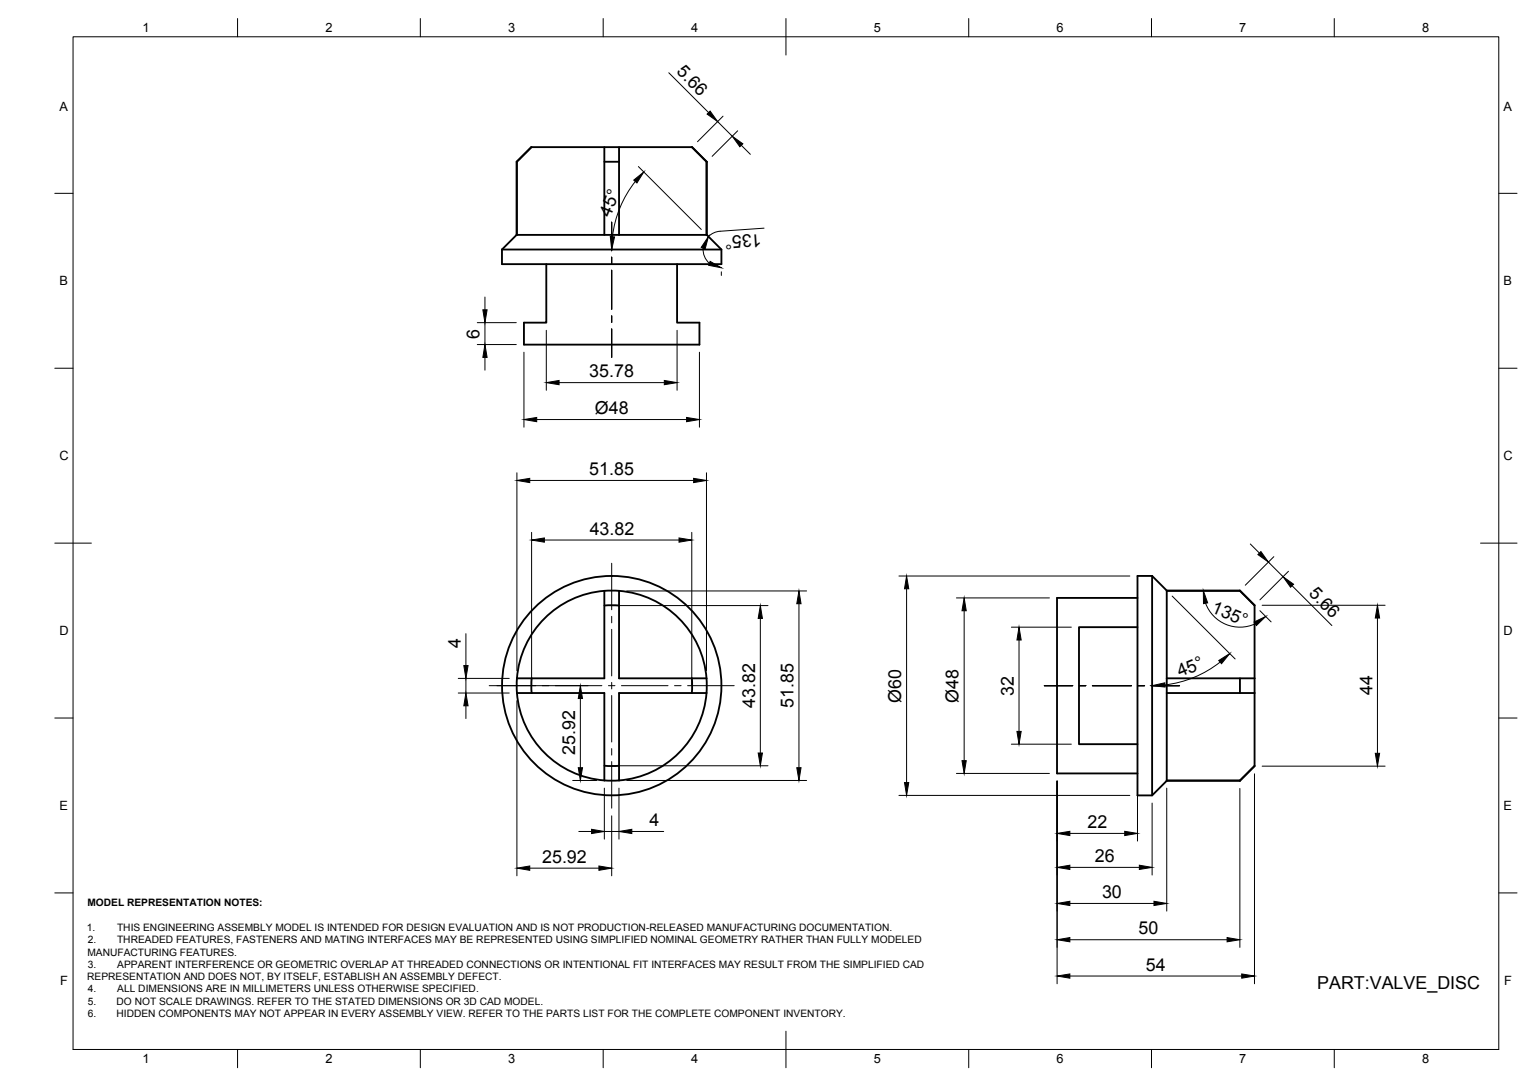
ISO-10303-21;
HEADER;
/* Generated by software containing ST-Developer
 * from STEP Tools, Inc. (www.steptools.com) 
 */

FILE_DESCRIPTION(
/* description */ (''),
/* implementation_level */ '2;1');

FILE_NAME(
/* name */ 'VALVE_DISC.step',
/* time_stamp */ '2026-10-04T02:10:06-07:00',
/* author */ (''),
/* organization */ (''),
/* preprocessor_version */ 'ST-DEVELOPER v20.2',
/* originating_system */ 'Autodesk Translation Framework v15.15.0.0',
/* authorisation */ '');

FILE_SCHEMA (('AUTOMOTIVE_DESIGN { 1 0 10303 214 3 1 1 }'));
ENDSEC;

DATA;
#10=MECHANICAL_DESIGN_GEOMETRIC_PRESENTATION_REPRESENTATION('',(#142),#9668);
#75=(
BOUNDED_CURVE()
B_SPLINE_CURVE(2,(#6291,#6292,#6293),.UNSPECIFIED.,.F.,.F.)
B_SPLINE_CURVE_WITH_KNOTS((3,3),(-0.968089558975317,-0.208236182755166),
 .UNSPECIFIED.)
CURVE()
GEOMETRIC_REPRESENTATION_ITEM()
RATIONAL_B_SPLINE_CURVE((1.03202593839996,1.02394290093172,1.00881846372195))
REPRESENTATION_ITEM('')
);
#76=(
BOUNDED_CURVE()
B_SPLINE_CURVE(2,(#6302,#6303,#6304),.UNSPECIFIED.,.F.,.F.)
B_SPLINE_CURVE_WITH_KNOTS((3,3),(-3.47246065490362,-2.71260727868867),
 .UNSPECIFIED.)
CURVE()
GEOMETRIC_REPRESENTATION_ITEM()
RATIONAL_B_SPLINE_CURVE((1.00881846372215,1.02394290093178,1.03202593839996))
REPRESENTATION_ITEM('')
);
#77=(
BOUNDED_CURVE()
B_SPLINE_CURVE(2,(#6312,#6313,#6314),.UNSPECIFIED.,.F.,.F.)
B_SPLINE_CURVE_WITH_KNOTS((3,3),(-3.47246065490362,-2.71260727868867),
 .UNSPECIFIED.)
CURVE()
GEOMETRIC_REPRESENTATION_ITEM()
RATIONAL_B_SPLINE_CURVE((1.00881846372215,1.02394290093178,1.03202593839996))
REPRESENTATION_ITEM('')
);
#78=(
BOUNDED_CURVE()
B_SPLINE_CURVE(2,(#6321,#6322,#6323),.UNSPECIFIED.,.F.,.F.)
B_SPLINE_CURVE_WITH_KNOTS((3,3),(-0.968089558975317,-0.208236182755166),
 .UNSPECIFIED.)
CURVE()
GEOMETRIC_REPRESENTATION_ITEM()
RATIONAL_B_SPLINE_CURVE((1.03202593839996,1.02394290093172,1.00881846372195))
REPRESENTATION_ITEM('')
);
#79=(
BOUNDED_CURVE()
B_SPLINE_CURVE(2,(#6399,#6400,#6401),.UNSPECIFIED.,.F.,.F.)
B_SPLINE_CURVE_WITH_KNOTS((3,3),(-3.47246065490413,-2.71260727868925),
 .UNSPECIFIED.)
CURVE()
GEOMETRIC_REPRESENTATION_ITEM()
RATIONAL_B_SPLINE_CURVE((1.00881846372252,1.0239429009328,1.03202593840134))
REPRESENTATION_ITEM('')
);
#80=(
BOUNDED_CURVE()
B_SPLINE_CURVE(2,(#6406,#6407,#6408),.UNSPECIFIED.,.F.,.F.)
B_SPLINE_CURVE_WITH_KNOTS((3,3),(-0.968089559028266,-0.20823618276597),
 .UNSPECIFIED.)
CURVE()
GEOMETRIC_REPRESENTATION_ITEM()
RATIONAL_B_SPLINE_CURVE((1.03202593842995,1.02394290095447,1.00881846373032))
REPRESENTATION_ITEM('')
);
#81=(
BOUNDED_CURVE()
B_SPLINE_CURVE(2,(#6413,#6414,#6415),.UNSPECIFIED.,.F.,.F.)
B_SPLINE_CURVE_WITH_KNOTS((3,3),(-3.47246065490413,-2.71260727868925),
 .UNSPECIFIED.)
CURVE()
GEOMETRIC_REPRESENTATION_ITEM()
RATIONAL_B_SPLINE_CURVE((1.00881846372251,1.0239429009328,1.03202593840134))
REPRESENTATION_ITEM('')
);
#82=(
BOUNDED_CURVE()
B_SPLINE_CURVE(2,(#6420,#6421,#6422),.UNSPECIFIED.,.F.,.F.)
B_SPLINE_CURVE_WITH_KNOTS((3,3),(-0.968089559028514,-0.208236182766157),
 .UNSPECIFIED.)
CURVE()
GEOMETRIC_REPRESENTATION_ITEM()
RATIONAL_B_SPLINE_CURVE((1.03202593842948,1.02394290095412,1.0088184637302))
REPRESENTATION_ITEM('')
);
#120=SHAPE_REPRESENTATION_RELATIONSHIP('SRR','None',#9713,#131);
#131=ADVANCED_BREP_SHAPE_REPRESENTATION('',(#153),#9658);
#142=STYLED_ITEM('',(#9775),#153);
#153=MANIFOLD_SOLID_BREP('Body1',#3882);
#165=CONICAL_SURFACE('',#4162,26.,0.785398163397448);
#166=CONICAL_SURFACE('',#4190,22.,0.785398163397446);
#167=CONICAL_SURFACE('',#4191,22.,0.785398163397446);
#168=CONICAL_SURFACE('',#4192,22.,0.785398163397446);
#169=CONICAL_SURFACE('',#4193,22.,0.785398163397446);
#229=FACE_BOUND('',#1124,.T.);
#230=FACE_BOUND('',#1127,.T.);
#231=FACE_BOUND('',#1128,.T.);
#232=FACE_BOUND('',#1133,.T.);
#281=PLANE('',#4136);
#282=PLANE('',#4138);
#283=PLANE('',#4140);
#284=PLANE('',#4142);
#285=PLANE('',#4144);
#286=PLANE('',#4145);
#287=PLANE('',#4146);
#288=PLANE('',#4147);
#289=PLANE('',#4148);
#290=PLANE('',#4157);
#291=PLANE('',#4168);
#292=PLANE('',#4169);
#293=PLANE('',#4171);
#294=PLANE('',#4177);
#295=PLANE('',#4182);
#296=PLANE('',#4183);
#297=PLANE('',#4186);
#298=PLANE('',#4187);
#406=LINE('',#6264,#597);
#407=LINE('',#6265,#598);
#408=LINE('',#6269,#599);
#409=LINE('',#6271,#600);
#410=LINE('',#6276,#601);
#411=LINE('',#6278,#602);
#412=LINE('',#6285,#603);
#413=LINE('',#6286,#604);
#414=LINE('',#6289,#605);
#415=LINE('',#6295,#606);
#416=LINE('',#6296,#607);
#417=LINE('',#6300,#608);
#418=LINE('',#6305,#609);
#419=LINE('',#6306,#610);
#420=LINE('',#6310,#611);
#421=LINE('',#6315,#612);
#422=LINE('',#6316,#613);
#423=LINE('',#6319,#614);
#424=LINE('',#6325,#615);
#425=LINE('',#6326,#616);
#426=LINE('',#6335,#617);
#427=LINE('',#6338,#618);
#428=LINE('',#6342,#619);
#429=LINE('',#6346,#620);
#430=LINE('',#6350,#621);
#431=LINE('',#6355,#622);
#432=LINE('',#6356,#623);
#433=LINE('',#6362,#624);
#434=LINE('',#6365,#625);
#435=LINE('',#6372,#626);
#436=LINE('',#6374,#627);
#437=LINE('',#6379,#628);
#438=LINE('',#6386,#629);
#439=LINE('',#6389,#630);
#440=LINE('',#6392,#631);
#441=LINE('',#6395,#632);
#442=LINE('',#6402,#633);
#443=LINE('',#6405,#634);
#444=LINE('',#6416,#635);
#445=LINE('',#6419,#636);
#597=VECTOR('',#4752,23.9229627936314);
#598=VECTOR('',#4753,23.9229627936314);
#599=VECTOR('',#4756,23.9229627936314);
#600=VECTOR('',#4757,23.9229627936314);
#601=VECTOR('',#4762,23.9229627936314);
#602=VECTOR('',#4763,23.9229627936314);
#603=VECTOR('',#4770,23.9229627936314);
#604=VECTOR('',#4771,23.9229627936314);
#605=VECTOR('',#4774,20.);
#606=VECTOR('',#4775,19.9089023002066);
#607=VECTOR('',#4776,24.);
#608=VECTOR('',#4779,19.9089023002066);
#609=VECTOR('',#4780,20.);
#610=VECTOR('',#4781,24.);
#611=VECTOR('',#4784,19.9089023002066);
#612=VECTOR('',#4785,20.);
#613=VECTOR('',#4786,24.);
#614=VECTOR('',#4789,20.);
#615=VECTOR('',#4790,19.9089023002066);
#616=VECTOR('',#4791,24.);
#617=VECTOR('',#4800,16.);
#618=VECTOR('',#4803,24.);
#619=VECTOR('',#4806,16.);
#620=VECTOR('',#4809,16.);
#621=VECTOR('',#4812,16.);
#622=VECTOR('',#4819,35.7770876399966);
#623=VECTOR('',#4820,35.7770876399966);
#624=VECTOR('',#4827,30.);
#625=VECTOR('',#4830,26.);
#626=VECTOR('',#4843,35.7770876399966);
#627=VECTOR('',#4846,35.7770876399966);
#628=VECTOR('',#4853,11.);
#629=VECTOR('',#4864,19.9089023002066);
#630=VECTOR('',#4867,19.9089023002066);
#631=VECTOR('',#4870,19.9089023002066);
#632=VECTOR('',#4873,19.9089023002066);
#633=VECTOR('',#4878,20.);
#634=VECTOR('',#4881,20.);
#635=VECTOR('',#4888,20.);
#636=VECTOR('',#4891,20.);
#779=CYLINDRICAL_SURFACE('',#4151,24.);
#780=CYLINDRICAL_SURFACE('',#4159,30.);
#781=CYLINDRICAL_SURFACE('',#4172,11.);
#782=CYLINDRICAL_SURFACE('',#4173,26.);
#783=CYLINDRICAL_SURFACE('',#4175,26.);
#784=CYLINDRICAL_SURFACE('',#4184,26.);
#785=CYLINDRICAL_SURFACE('',#4188,26.);
#858=FACE_OUTER_BOUND('',#1115,.T.);
#859=FACE_OUTER_BOUND('',#1116,.T.);
#860=FACE_OUTER_BOUND('',#1117,.T.);
#861=FACE_OUTER_BOUND('',#1118,.T.);
#862=FACE_OUTER_BOUND('',#1119,.T.);
#863=FACE_OUTER_BOUND('',#1120,.T.);
#864=FACE_OUTER_BOUND('',#1121,.T.);
#865=FACE_OUTER_BOUND('',#1122,.T.);
#866=FACE_OUTER_BOUND('',#1123,.T.);
#867=FACE_OUTER_BOUND('',#1125,.T.);
#868=FACE_OUTER_BOUND('',#1126,.T.);
#869=FACE_OUTER_BOUND('',#1129,.T.);
#870=FACE_OUTER_BOUND('',#1130,.T.);
#871=FACE_OUTER_BOUND('',#1131,.T.);
#872=FACE_OUTER_BOUND('',#1132,.T.);
#873=FACE_OUTER_BOUND('',#1134,.T.);
#874=FACE_OUTER_BOUND('',#1135,.T.);
#875=FACE_OUTER_BOUND('',#1136,.T.);
#876=FACE_OUTER_BOUND('',#1137,.T.);
#877=FACE_OUTER_BOUND('',#1138,.T.);
#878=FACE_OUTER_BOUND('',#1139,.T.);
#879=FACE_OUTER_BOUND('',#1140,.T.);
#880=FACE_OUTER_BOUND('',#1141,.T.);
#881=FACE_OUTER_BOUND('',#1142,.T.);
#882=FACE_OUTER_BOUND('',#1143,.T.);
#883=FACE_OUTER_BOUND('',#1144,.T.);
#884=FACE_OUTER_BOUND('',#1145,.T.);
#885=FACE_OUTER_BOUND('',#1146,.T.);
#886=FACE_OUTER_BOUND('',#1147,.T.);
#887=FACE_OUTER_BOUND('',#1148,.T.);
#1115=EDGE_LOOP('',(#2781,#2782,#2783));
#1116=EDGE_LOOP('',(#2784,#2785,#2786));
#1117=EDGE_LOOP('',(#2787,#2788,#2789));
#1118=EDGE_LOOP('',(#2790,#2791,#2792));
#1119=EDGE_LOOP('',(#2793,#2794,#2795,#2796,#2797));
#1120=EDGE_LOOP('',(#2798,#2799,#2800,#2801,#2802));
#1121=EDGE_LOOP('',(#2803,#2804,#2805,#2806,#2807));
#1122=EDGE_LOOP('',(#2808,#2809,#2810,#2811,#2812));
#1123=EDGE_LOOP('',(#2813));
#1124=EDGE_LOOP('',(#2814));
#1125=EDGE_LOOP('',(#2815,#2816,#2817,#2818,#2819,#2820,#2821,#2822,#2823,
#2824,#2825,#2826));
#1126=EDGE_LOOP('',(#2827));
#1127=EDGE_LOOP('',(#2828,#2829));
#1128=EDGE_LOOP('',(#2830,#2831));
#1129=EDGE_LOOP('',(#2832,#2833,#2834,#2835,#2836));
#1130=EDGE_LOOP('',(#2837,#2838,#2839,#2840,#2841,#2842,#2843,#2844,#2845,
#2846,#2847,#2848,#2849));
#1131=EDGE_LOOP('',(#2850,#2851,#2852,#2853));
#1132=EDGE_LOOP('',(#2854,#2855,#2856,#2857,#2858));
#1133=EDGE_LOOP('',(#2859));
#1134=EDGE_LOOP('',(#2860,#2861,#2862,#2863));
#1135=EDGE_LOOP('',(#2864,#2865,#2866,#2867));
#1136=EDGE_LOOP('',(#2868,#2869,#2870,#2871));
#1137=EDGE_LOOP('',(#2872,#2873,#2874,#2875));
#1138=EDGE_LOOP('',(#2876,#2877,#2878,#2879,#2880,#2881,#2882,#2883,#2884,
#2885,#2886,#2887));
#1139=EDGE_LOOP('',(#2888,#2889,#2890,#2891,#2892));
#1140=EDGE_LOOP('',(#2893,#2894,#2895,#2896,#2897));
#1141=EDGE_LOOP('',(#2898,#2899,#2900,#2901,#2902));
#1142=EDGE_LOOP('',(#2903,#2904,#2905,#2906,#2907));
#1143=EDGE_LOOP('',(#2908,#2909,#2910,#2911,#2912));
#1144=EDGE_LOOP('',(#2913,#2914,#2915,#2916));
#1145=EDGE_LOOP('',(#2917,#2918,#2919,#2920));
#1146=EDGE_LOOP('',(#2921,#2922,#2923,#2924));
#1147=EDGE_LOOP('',(#2925,#2926,#2927,#2928));
#1148=EDGE_LOOP('',(#2929,#2930,#2931,#2932));
#1498=CIRCLE('',#4137,26.);
#1499=CIRCLE('',#4139,26.);
#1500=CIRCLE('',#4141,26.);
#1501=CIRCLE('',#4143,26.);
#1502=CIRCLE('',#4149,24.);
#1503=CIRCLE('',#4150,11.);
#1504=CIRCLE('',#4152,24.);
#1505=CIRCLE('',#4153,24.);
#1506=CIRCLE('',#4154,24.);
#1507=CIRCLE('',#4155,24.);
#1508=CIRCLE('',#4156,24.);
#1509=CIRCLE('',#4158,30.);
#1510=CIRCLE('',#4160,30.);
#1511=CIRCLE('',#4161,30.);
#1512=CIRCLE('',#4163,26.);
#1513=CIRCLE('',#4164,26.);
#1514=CIRCLE('',#4165,26.);
#1515=CIRCLE('',#4166,26.);
#1516=CIRCLE('',#4167,26.);
#1517=CIRCLE('',#4170,11.);
#1518=CIRCLE('',#4174,26.);
#1519=CIRCLE('',#4176,26.);
#1520=CIRCLE('',#4178,22.);
#1521=CIRCLE('',#4179,22.);
#1522=CIRCLE('',#4180,22.);
#1523=CIRCLE('',#4181,22.);
#1524=CIRCLE('',#4185,26.);
#1525=CIRCLE('',#4189,26.);
#1721=VERTEX_POINT('',#6260);
#1722=VERTEX_POINT('',#6261);
#1723=VERTEX_POINT('',#6263);
#1724=VERTEX_POINT('',#6267);
#1725=VERTEX_POINT('',#6268);
#1726=VERTEX_POINT('',#6270);
#1727=VERTEX_POINT('',#6274);
#1728=VERTEX_POINT('',#6275);
#1729=VERTEX_POINT('',#6277);
#1730=VERTEX_POINT('',#6281);
#1731=VERTEX_POINT('',#6282);
#1732=VERTEX_POINT('',#6284);
#1733=VERTEX_POINT('',#6288);
#1734=VERTEX_POINT('',#6290);
#1735=VERTEX_POINT('',#6294);
#1736=VERTEX_POINT('',#6298);
#1737=VERTEX_POINT('',#6299);
#1738=VERTEX_POINT('',#6301);
#1739=VERTEX_POINT('',#6308);
#1740=VERTEX_POINT('',#6309);
#1741=VERTEX_POINT('',#6311);
#1742=VERTEX_POINT('',#6318);
#1743=VERTEX_POINT('',#6320);
#1744=VERTEX_POINT('',#6324);
#1745=VERTEX_POINT('',#6328);
#1746=VERTEX_POINT('',#6330);
#1747=VERTEX_POINT('',#6333);
#1748=VERTEX_POINT('',#6334);
#1749=VERTEX_POINT('',#6336);
#1750=VERTEX_POINT('',#6339);
#1751=VERTEX_POINT('',#6341);
#1752=VERTEX_POINT('',#6343);
#1753=VERTEX_POINT('',#6345);
#1754=VERTEX_POINT('',#6347);
#1755=VERTEX_POINT('',#6349);
#1756=VERTEX_POINT('',#6353);
#1757=VERTEX_POINT('',#6358);
#1758=VERTEX_POINT('',#6359);
#1759=VERTEX_POINT('',#6364);
#1760=VERTEX_POINT('',#6375);
#1761=VERTEX_POINT('',#6385);
#1762=VERTEX_POINT('',#6387);
#1763=VERTEX_POINT('',#6391);
#1764=VERTEX_POINT('',#6393);
#1765=VERTEX_POINT('',#6398);
#1766=VERTEX_POINT('',#6404);
#1767=VERTEX_POINT('',#6412);
#1768=VERTEX_POINT('',#6418);
#2114=EDGE_CURVE('',#1721,#1722,#1498,.T.);
#2115=EDGE_CURVE('',#1723,#1722,#406,.T.);
#2116=EDGE_CURVE('',#1721,#1723,#407,.T.);
#2117=EDGE_CURVE('',#1724,#1725,#408,.T.);
#2118=EDGE_CURVE('',#1726,#1724,#409,.T.);
#2119=EDGE_CURVE('',#1726,#1725,#1499,.T.);
#2120=EDGE_CURVE('',#1727,#1728,#410,.T.);
#2121=EDGE_CURVE('',#1729,#1727,#411,.T.);
#2122=EDGE_CURVE('',#1729,#1728,#1500,.T.);
#2123=EDGE_CURVE('',#1730,#1731,#1501,.T.);
#2124=EDGE_CURVE('',#1732,#1731,#412,.T.);
#2125=EDGE_CURVE('',#1730,#1732,#413,.T.);
#2126=EDGE_CURVE('',#1733,#1728,#414,.T.);
#2127=EDGE_CURVE('',#1733,#1734,#75,.T.);
#2128=EDGE_CURVE('',#1735,#1734,#415,.T.);
#2129=EDGE_CURVE('',#1727,#1735,#416,.T.);
#2130=EDGE_CURVE('',#1736,#1737,#417,.T.);
#2131=EDGE_CURVE('',#1736,#1738,#76,.T.);
#2132=EDGE_CURVE('',#1738,#1730,#418,.T.);
#2133=EDGE_CURVE('',#1737,#1732,#419,.T.);
#2134=EDGE_CURVE('',#1739,#1740,#420,.T.);
#2135=EDGE_CURVE('',#1739,#1741,#77,.T.);
#2136=EDGE_CURVE('',#1741,#1721,#421,.T.);
#2137=EDGE_CURVE('',#1740,#1723,#422,.T.);
#2138=EDGE_CURVE('',#1742,#1725,#423,.T.);
#2139=EDGE_CURVE('',#1742,#1743,#78,.T.);
#2140=EDGE_CURVE('',#1744,#1743,#424,.T.);
#2141=EDGE_CURVE('',#1724,#1744,#425,.T.);
#2142=EDGE_CURVE('',#1745,#1745,#1502,.T.);
#2143=EDGE_CURVE('',#1746,#1746,#1503,.F.);
#2144=EDGE_CURVE('',#1747,#1748,#426,.T.);
#2145=EDGE_CURVE('',#1749,#1747,#1504,.F.);
#2146=EDGE_CURVE('',#1749,#1745,#427,.T.);
#2147=EDGE_CURVE('',#1750,#1749,#1505,.F.);
#2148=EDGE_CURVE('',#1751,#1750,#428,.F.);
#2149=EDGE_CURVE('',#1752,#1751,#1506,.T.);
#2150=EDGE_CURVE('',#1753,#1752,#429,.T.);
#2151=EDGE_CURVE('',#1754,#1753,#1507,.F.);
#2152=EDGE_CURVE('',#1755,#1754,#430,.F.);
#2153=EDGE_CURVE('',#1748,#1755,#1508,.T.);
#2154=EDGE_CURVE('',#1756,#1756,#1509,.T.);
#2155=EDGE_CURVE('',#1752,#1751,#431,.T.);
#2156=EDGE_CURVE('',#1755,#1748,#432,.T.);
#2157=EDGE_CURVE('',#1757,#1758,#1510,.T.);
#2158=EDGE_CURVE('',#1758,#1757,#1511,.T.);
#2159=EDGE_CURVE('',#1758,#1756,#433,.T.);
#2160=EDGE_CURVE('',#1757,#1759,#434,.T.);
#2161=EDGE_CURVE('',#1722,#1759,#1512,.T.);
#2162=EDGE_CURVE('',#1728,#1721,#1513,.T.);
#2163=EDGE_CURVE('',#1731,#1729,#1514,.T.);
#2164=EDGE_CURVE('',#1725,#1730,#1515,.T.);
#2165=EDGE_CURVE('',#1759,#1726,#1516,.T.);
#2166=EDGE_CURVE('',#1754,#1747,#435,.T.);
#2167=EDGE_CURVE('',#1753,#1750,#436,.T.);
#2168=EDGE_CURVE('',#1760,#1760,#1517,.F.);
#2169=EDGE_CURVE('',#1746,#1760,#437,.T.);
#2170=EDGE_CURVE('',#1738,#1742,#1518,.F.);
#2171=EDGE_CURVE('',#1741,#1733,#1519,.F.);
#2172=EDGE_CURVE('',#1737,#1761,#438,.T.);
#2173=EDGE_CURVE('',#1761,#1762,#1520,.T.);
#2174=EDGE_CURVE('',#1762,#1735,#439,.T.);
#2175=EDGE_CURVE('',#1734,#1739,#1521,.T.);
#2176=EDGE_CURVE('',#1740,#1763,#440,.T.);
#2177=EDGE_CURVE('',#1763,#1764,#1522,.T.);
#2178=EDGE_CURVE('',#1764,#1744,#441,.T.);
#2179=EDGE_CURVE('',#1743,#1736,#1523,.T.);
#2180=EDGE_CURVE('',#1764,#1765,#79,.T.);
#2181=EDGE_CURVE('',#1765,#1726,#442,.T.);
#2182=EDGE_CURVE('',#1766,#1722,#443,.T.);
#2183=EDGE_CURVE('',#1766,#1763,#80,.T.);
#2184=EDGE_CURVE('',#1765,#1766,#1524,.F.);
#2185=EDGE_CURVE('',#1762,#1767,#81,.T.);
#2186=EDGE_CURVE('',#1767,#1729,#444,.T.);
#2187=EDGE_CURVE('',#1768,#1731,#445,.T.);
#2188=EDGE_CURVE('',#1768,#1761,#82,.T.);
#2189=EDGE_CURVE('',#1767,#1768,#1525,.F.);
#2781=ORIENTED_EDGE('',*,*,#2114,.T.);
#2782=ORIENTED_EDGE('',*,*,#2115,.F.);
#2783=ORIENTED_EDGE('',*,*,#2116,.F.);
#2784=ORIENTED_EDGE('',*,*,#2117,.F.);
#2785=ORIENTED_EDGE('',*,*,#2118,.F.);
#2786=ORIENTED_EDGE('',*,*,#2119,.T.);
#2787=ORIENTED_EDGE('',*,*,#2120,.F.);
#2788=ORIENTED_EDGE('',*,*,#2121,.F.);
#2789=ORIENTED_EDGE('',*,*,#2122,.T.);
#2790=ORIENTED_EDGE('',*,*,#2123,.T.);
#2791=ORIENTED_EDGE('',*,*,#2124,.F.);
#2792=ORIENTED_EDGE('',*,*,#2125,.F.);
#2793=ORIENTED_EDGE('',*,*,#2126,.F.);
#2794=ORIENTED_EDGE('',*,*,#2127,.T.);
#2795=ORIENTED_EDGE('',*,*,#2128,.F.);
#2796=ORIENTED_EDGE('',*,*,#2129,.F.);
#2797=ORIENTED_EDGE('',*,*,#2120,.T.);
#2798=ORIENTED_EDGE('',*,*,#2130,.F.);
#2799=ORIENTED_EDGE('',*,*,#2131,.T.);
#2800=ORIENTED_EDGE('',*,*,#2132,.T.);
#2801=ORIENTED_EDGE('',*,*,#2125,.T.);
#2802=ORIENTED_EDGE('',*,*,#2133,.F.);
#2803=ORIENTED_EDGE('',*,*,#2134,.F.);
#2804=ORIENTED_EDGE('',*,*,#2135,.T.);
#2805=ORIENTED_EDGE('',*,*,#2136,.T.);
#2806=ORIENTED_EDGE('',*,*,#2116,.T.);
#2807=ORIENTED_EDGE('',*,*,#2137,.F.);
#2808=ORIENTED_EDGE('',*,*,#2138,.F.);
#2809=ORIENTED_EDGE('',*,*,#2139,.T.);
#2810=ORIENTED_EDGE('',*,*,#2140,.F.);
#2811=ORIENTED_EDGE('',*,*,#2141,.F.);
#2812=ORIENTED_EDGE('',*,*,#2117,.T.);
#2813=ORIENTED_EDGE('',*,*,#2142,.F.);
#2814=ORIENTED_EDGE('',*,*,#2143,.T.);
#2815=ORIENTED_EDGE('',*,*,#2144,.F.);
#2816=ORIENTED_EDGE('',*,*,#2145,.F.);
#2817=ORIENTED_EDGE('',*,*,#2146,.T.);
#2818=ORIENTED_EDGE('',*,*,#2142,.T.);
#2819=ORIENTED_EDGE('',*,*,#2146,.F.);
#2820=ORIENTED_EDGE('',*,*,#2147,.F.);
#2821=ORIENTED_EDGE('',*,*,#2148,.F.);
#2822=ORIENTED_EDGE('',*,*,#2149,.F.);
#2823=ORIENTED_EDGE('',*,*,#2150,.F.);
#2824=ORIENTED_EDGE('',*,*,#2151,.F.);
#2825=ORIENTED_EDGE('',*,*,#2152,.F.);
#2826=ORIENTED_EDGE('',*,*,#2153,.F.);
#2827=ORIENTED_EDGE('',*,*,#2154,.F.);
#2828=ORIENTED_EDGE('',*,*,#2149,.T.);
#2829=ORIENTED_EDGE('',*,*,#2155,.F.);
#2830=ORIENTED_EDGE('',*,*,#2153,.T.);
#2831=ORIENTED_EDGE('',*,*,#2156,.T.);
#2832=ORIENTED_EDGE('',*,*,#2157,.F.);
#2833=ORIENTED_EDGE('',*,*,#2158,.F.);
#2834=ORIENTED_EDGE('',*,*,#2159,.T.);
#2835=ORIENTED_EDGE('',*,*,#2154,.T.);
#2836=ORIENTED_EDGE('',*,*,#2159,.F.);
#2837=ORIENTED_EDGE('',*,*,#2157,.T.);
#2838=ORIENTED_EDGE('',*,*,#2158,.T.);
#2839=ORIENTED_EDGE('',*,*,#2160,.T.);
#2840=ORIENTED_EDGE('',*,*,#2161,.F.);
#2841=ORIENTED_EDGE('',*,*,#2114,.F.);
#2842=ORIENTED_EDGE('',*,*,#2162,.F.);
#2843=ORIENTED_EDGE('',*,*,#2122,.F.);
#2844=ORIENTED_EDGE('',*,*,#2163,.F.);
#2845=ORIENTED_EDGE('',*,*,#2123,.F.);
#2846=ORIENTED_EDGE('',*,*,#2164,.F.);
#2847=ORIENTED_EDGE('',*,*,#2119,.F.);
#2848=ORIENTED_EDGE('',*,*,#2165,.F.);
#2849=ORIENTED_EDGE('',*,*,#2160,.F.);
#2850=ORIENTED_EDGE('',*,*,#2152,.T.);
#2851=ORIENTED_EDGE('',*,*,#2166,.T.);
#2852=ORIENTED_EDGE('',*,*,#2144,.T.);
#2853=ORIENTED_EDGE('',*,*,#2156,.F.);
#2854=ORIENTED_EDGE('',*,*,#2151,.T.);
#2855=ORIENTED_EDGE('',*,*,#2167,.T.);
#2856=ORIENTED_EDGE('',*,*,#2147,.T.);
#2857=ORIENTED_EDGE('',*,*,#2145,.T.);
#2858=ORIENTED_EDGE('',*,*,#2166,.F.);
#2859=ORIENTED_EDGE('',*,*,#2168,.F.);
#2860=ORIENTED_EDGE('',*,*,#2148,.T.);
#2861=ORIENTED_EDGE('',*,*,#2167,.F.);
#2862=ORIENTED_EDGE('',*,*,#2150,.T.);
#2863=ORIENTED_EDGE('',*,*,#2155,.T.);
#2864=ORIENTED_EDGE('',*,*,#2143,.F.);
#2865=ORIENTED_EDGE('',*,*,#2169,.T.);
#2866=ORIENTED_EDGE('',*,*,#2168,.T.);
#2867=ORIENTED_EDGE('',*,*,#2169,.F.);
#2868=ORIENTED_EDGE('',*,*,#2132,.F.);
#2869=ORIENTED_EDGE('',*,*,#2170,.T.);
#2870=ORIENTED_EDGE('',*,*,#2138,.T.);
#2871=ORIENTED_EDGE('',*,*,#2164,.T.);
#2872=ORIENTED_EDGE('',*,*,#2136,.F.);
#2873=ORIENTED_EDGE('',*,*,#2171,.T.);
#2874=ORIENTED_EDGE('',*,*,#2126,.T.);
#2875=ORIENTED_EDGE('',*,*,#2162,.T.);
#2876=ORIENTED_EDGE('',*,*,#2172,.T.);
#2877=ORIENTED_EDGE('',*,*,#2173,.T.);
#2878=ORIENTED_EDGE('',*,*,#2174,.T.);
#2879=ORIENTED_EDGE('',*,*,#2128,.T.);
#2880=ORIENTED_EDGE('',*,*,#2175,.T.);
#2881=ORIENTED_EDGE('',*,*,#2134,.T.);
#2882=ORIENTED_EDGE('',*,*,#2176,.T.);
#2883=ORIENTED_EDGE('',*,*,#2177,.T.);
#2884=ORIENTED_EDGE('',*,*,#2178,.T.);
#2885=ORIENTED_EDGE('',*,*,#2140,.T.);
#2886=ORIENTED_EDGE('',*,*,#2179,.T.);
#2887=ORIENTED_EDGE('',*,*,#2130,.T.);
#2888=ORIENTED_EDGE('',*,*,#2178,.F.);
#2889=ORIENTED_EDGE('',*,*,#2180,.T.);
#2890=ORIENTED_EDGE('',*,*,#2181,.T.);
#2891=ORIENTED_EDGE('',*,*,#2118,.T.);
#2892=ORIENTED_EDGE('',*,*,#2141,.T.);
#2893=ORIENTED_EDGE('',*,*,#2182,.F.);
#2894=ORIENTED_EDGE('',*,*,#2183,.T.);
#2895=ORIENTED_EDGE('',*,*,#2176,.F.);
#2896=ORIENTED_EDGE('',*,*,#2137,.T.);
#2897=ORIENTED_EDGE('',*,*,#2115,.T.);
#2898=ORIENTED_EDGE('',*,*,#2181,.F.);
#2899=ORIENTED_EDGE('',*,*,#2184,.T.);
#2900=ORIENTED_EDGE('',*,*,#2182,.T.);
#2901=ORIENTED_EDGE('',*,*,#2161,.T.);
#2902=ORIENTED_EDGE('',*,*,#2165,.T.);
#2903=ORIENTED_EDGE('',*,*,#2174,.F.);
#2904=ORIENTED_EDGE('',*,*,#2185,.T.);
#2905=ORIENTED_EDGE('',*,*,#2186,.T.);
#2906=ORIENTED_EDGE('',*,*,#2121,.T.);
#2907=ORIENTED_EDGE('',*,*,#2129,.T.);
#2908=ORIENTED_EDGE('',*,*,#2187,.F.);
#2909=ORIENTED_EDGE('',*,*,#2188,.T.);
#2910=ORIENTED_EDGE('',*,*,#2172,.F.);
#2911=ORIENTED_EDGE('',*,*,#2133,.T.);
#2912=ORIENTED_EDGE('',*,*,#2124,.T.);
#2913=ORIENTED_EDGE('',*,*,#2186,.F.);
#2914=ORIENTED_EDGE('',*,*,#2189,.T.);
#2915=ORIENTED_EDGE('',*,*,#2187,.T.);
#2916=ORIENTED_EDGE('',*,*,#2163,.T.);
#2917=ORIENTED_EDGE('',*,*,#2188,.F.);
#2918=ORIENTED_EDGE('',*,*,#2189,.F.);
#2919=ORIENTED_EDGE('',*,*,#2185,.F.);
#2920=ORIENTED_EDGE('',*,*,#2173,.F.);
#2921=ORIENTED_EDGE('',*,*,#2139,.F.);
#2922=ORIENTED_EDGE('',*,*,#2170,.F.);
#2923=ORIENTED_EDGE('',*,*,#2131,.F.);
#2924=ORIENTED_EDGE('',*,*,#2179,.F.);
#2925=ORIENTED_EDGE('',*,*,#2183,.F.);
#2926=ORIENTED_EDGE('',*,*,#2184,.F.);
#2927=ORIENTED_EDGE('',*,*,#2180,.F.);
#2928=ORIENTED_EDGE('',*,*,#2177,.F.);
#2929=ORIENTED_EDGE('',*,*,#2127,.F.);
#2930=ORIENTED_EDGE('',*,*,#2171,.F.);
#2931=ORIENTED_EDGE('',*,*,#2135,.F.);
#2932=ORIENTED_EDGE('',*,*,#2175,.F.);
#3706=ADVANCED_FACE('',(#858),#281,.T.);
#3707=ADVANCED_FACE('',(#859),#282,.T.);
#3708=ADVANCED_FACE('',(#860),#283,.T.);
#3709=ADVANCED_FACE('',(#861),#284,.T.);
#3710=ADVANCED_FACE('',(#862),#285,.F.);
#3711=ADVANCED_FACE('',(#863),#286,.F.);
#3712=ADVANCED_FACE('',(#864),#287,.F.);
#3713=ADVANCED_FACE('',(#865),#288,.F.);
#3714=ADVANCED_FACE('',(#866,#229),#289,.T.);
#3715=ADVANCED_FACE('',(#867),#779,.T.);
#3716=ADVANCED_FACE('',(#868,#230,#231),#290,.T.);
#3717=ADVANCED_FACE('',(#869),#780,.T.);
#3718=ADVANCED_FACE('',(#870),#165,.T.);
#3719=ADVANCED_FACE('',(#871),#291,.F.);
#3720=ADVANCED_FACE('',(#872,#232),#292,.F.);
#3721=ADVANCED_FACE('',(#873),#293,.F.);
#3722=ADVANCED_FACE('',(#874),#781,.F.);
#3723=ADVANCED_FACE('',(#875),#782,.T.);
#3724=ADVANCED_FACE('',(#876),#783,.T.);
#3725=ADVANCED_FACE('',(#877),#294,.T.);
#3726=ADVANCED_FACE('',(#878),#295,.F.);
#3727=ADVANCED_FACE('',(#879),#296,.F.);
#3728=ADVANCED_FACE('',(#880),#784,.T.);
#3729=ADVANCED_FACE('',(#881),#297,.F.);
#3730=ADVANCED_FACE('',(#882),#298,.F.);
#3731=ADVANCED_FACE('',(#883),#785,.T.);
#3732=ADVANCED_FACE('',(#884),#166,.T.);
#3733=ADVANCED_FACE('',(#885),#167,.T.);
#3734=ADVANCED_FACE('',(#886),#168,.T.);
#3735=ADVANCED_FACE('',(#887),#169,.T.);
#3882=CLOSED_SHELL('',(#3706,#3707,#3708,#3709,#3710,#3711,#3712,#3713,
#3714,#3715,#3716,#3717,#3718,#3719,#3720,#3721,#3722,#3723,#3724,#3725,
#3726,#3727,#3728,#3729,#3730,#3731,#3732,#3733,#3734,#3735));
#4135=AXIS2_PLACEMENT_3D('',#6258,#4746,#4747);
#4136=AXIS2_PLACEMENT_3D('',#6259,#4748,#4749);
#4137=AXIS2_PLACEMENT_3D('',#6262,#4750,#4751);
#4138=AXIS2_PLACEMENT_3D('',#6266,#4754,#4755);
#4139=AXIS2_PLACEMENT_3D('',#6272,#4758,#4759);
#4140=AXIS2_PLACEMENT_3D('',#6273,#4760,#4761);
#4141=AXIS2_PLACEMENT_3D('',#6279,#4764,#4765);
#4142=AXIS2_PLACEMENT_3D('',#6280,#4766,#4767);
#4143=AXIS2_PLACEMENT_3D('',#6283,#4768,#4769);
#4144=AXIS2_PLACEMENT_3D('',#6287,#4772,#4773);
#4145=AXIS2_PLACEMENT_3D('',#6297,#4777,#4778);
#4146=AXIS2_PLACEMENT_3D('',#6307,#4782,#4783);
#4147=AXIS2_PLACEMENT_3D('',#6317,#4787,#4788);
#4148=AXIS2_PLACEMENT_3D('',#6327,#4792,#4793);
#4149=AXIS2_PLACEMENT_3D('',#6329,#4794,#4795);
#4150=AXIS2_PLACEMENT_3D('',#6331,#4796,#4797);
#4151=AXIS2_PLACEMENT_3D('',#6332,#4798,#4799);
#4152=AXIS2_PLACEMENT_3D('',#6337,#4801,#4802);
#4153=AXIS2_PLACEMENT_3D('',#6340,#4804,#4805);
#4154=AXIS2_PLACEMENT_3D('',#6344,#4807,#4808);
#4155=AXIS2_PLACEMENT_3D('',#6348,#4810,#4811);
#4156=AXIS2_PLACEMENT_3D('',#6351,#4813,#4814);
#4157=AXIS2_PLACEMENT_3D('',#6352,#4815,#4816);
#4158=AXIS2_PLACEMENT_3D('',#6354,#4817,#4818);
#4159=AXIS2_PLACEMENT_3D('',#6357,#4821,#4822);
#4160=AXIS2_PLACEMENT_3D('',#6360,#4823,#4824);
#4161=AXIS2_PLACEMENT_3D('',#6361,#4825,#4826);
#4162=AXIS2_PLACEMENT_3D('',#6363,#4828,#4829);
#4163=AXIS2_PLACEMENT_3D('',#6366,#4831,#4832);
#4164=AXIS2_PLACEMENT_3D('',#6367,#4833,#4834);
#4165=AXIS2_PLACEMENT_3D('',#6368,#4835,#4836);
#4166=AXIS2_PLACEMENT_3D('',#6369,#4837,#4838);
#4167=AXIS2_PLACEMENT_3D('',#6370,#4839,#4840);
#4168=AXIS2_PLACEMENT_3D('',#6371,#4841,#4842);
#4169=AXIS2_PLACEMENT_3D('',#6373,#4844,#4845);
#4170=AXIS2_PLACEMENT_3D('',#6376,#4847,#4848);
#4171=AXIS2_PLACEMENT_3D('',#6377,#4849,#4850);
#4172=AXIS2_PLACEMENT_3D('',#6378,#4851,#4852);
#4173=AXIS2_PLACEMENT_3D('',#6380,#4854,#4855);
#4174=AXIS2_PLACEMENT_3D('',#6381,#4856,#4857);
#4175=AXIS2_PLACEMENT_3D('',#6382,#4858,#4859);
#4176=AXIS2_PLACEMENT_3D('',#6383,#4860,#4861);
#4177=AXIS2_PLACEMENT_3D('',#6384,#4862,#4863);
#4178=AXIS2_PLACEMENT_3D('',#6388,#4865,#4866);
#4179=AXIS2_PLACEMENT_3D('',#6390,#4868,#4869);
#4180=AXIS2_PLACEMENT_3D('',#6394,#4871,#4872);
#4181=AXIS2_PLACEMENT_3D('',#6396,#4874,#4875);
#4182=AXIS2_PLACEMENT_3D('',#6397,#4876,#4877);
#4183=AXIS2_PLACEMENT_3D('',#6403,#4879,#4880);
#4184=AXIS2_PLACEMENT_3D('',#6409,#4882,#4883);
#4185=AXIS2_PLACEMENT_3D('',#6410,#4884,#4885);
#4186=AXIS2_PLACEMENT_3D('',#6411,#4886,#4887);
#4187=AXIS2_PLACEMENT_3D('',#6417,#4889,#4890);
#4188=AXIS2_PLACEMENT_3D('',#6423,#4892,#4893);
#4189=AXIS2_PLACEMENT_3D('',#6424,#4894,#4895);
#4190=AXIS2_PLACEMENT_3D('',#6425,#4896,#4897);
#4191=AXIS2_PLACEMENT_3D('',#6426,#4898,#4899);
#4192=AXIS2_PLACEMENT_3D('',#6427,#4900,#4901);
#4193=AXIS2_PLACEMENT_3D('',#6428,#4902,#4903);
#4746=DIRECTION('axis',(0.,0.,1.));
#4747=DIRECTION('refdir',(1.,0.,0.));
#4748=DIRECTION('center_axis',(0.,-1.,0.));
#4749=DIRECTION('ref_axis',(0.,0.,-1.));
#4750=DIRECTION('center_axis',(0.,-1.,0.));
#4751=DIRECTION('ref_axis',(0.,0.,-1.));
#4752=DIRECTION('',(3.50382346376903E-15,0.,-1.));
#4753=DIRECTION('',(1.,0.,0.));
#4754=DIRECTION('center_axis',(0.,-1.,0.));
#4755=DIRECTION('ref_axis',(0.,0.,-1.));
#4756=DIRECTION('',(1.,0.,0.));
#4757=DIRECTION('',(-3.49222139931946E-15,0.,1.));
#4758=DIRECTION('center_axis',(0.,-1.,0.));
#4759=DIRECTION('ref_axis',(0.,0.,-1.));
#4760=DIRECTION('center_axis',(0.,-1.,0.));
#4761=DIRECTION('ref_axis',(0.,0.,-1.));
#4762=DIRECTION('',(-1.,0.,0.));
#4763=DIRECTION('',(3.4806193348699E-15,0.,-1.));
#4764=DIRECTION('center_axis',(0.,-1.,0.));
#4765=DIRECTION('ref_axis',(0.,0.,-1.));
#4766=DIRECTION('center_axis',(0.,-1.,0.));
#4767=DIRECTION('ref_axis',(0.,0.,-1.));
#4768=DIRECTION('center_axis',(0.,-1.,0.));
#4769=DIRECTION('ref_axis',(0.,0.,-1.));
#4770=DIRECTION('',(-3.4806193348699E-15,0.,1.));
#4771=DIRECTION('',(-1.,0.,0.));
#4772=DIRECTION('center_axis',(0.,0.,-1.));
#4773=DIRECTION('ref_axis',(-1.,0.,0.));
#4774=DIRECTION('',(0.,1.,0.));
#4775=DIRECTION('',(-1.,0.,0.));
#4776=DIRECTION('',(0.,-1.,0.));
#4777=DIRECTION('center_axis',(0.,0.,-1.));
#4778=DIRECTION('ref_axis',(-1.,0.,0.));
#4779=DIRECTION('',(-1.,0.,0.));
#4780=DIRECTION('',(0.,1.,0.));
#4781=DIRECTION('',(0.,1.,0.));
#4782=DIRECTION('center_axis',(0.,0.,1.));
#4783=DIRECTION('ref_axis',(1.,0.,0.));
#4784=DIRECTION('',(1.,0.,0.));
#4785=DIRECTION('',(0.,1.,0.));
#4786=DIRECTION('',(0.,1.,0.));
#4787=DIRECTION('center_axis',(0.,0.,1.));
#4788=DIRECTION('ref_axis',(1.,0.,0.));
#4789=DIRECTION('',(0.,1.,0.));
#4790=DIRECTION('',(1.,0.,0.));
#4791=DIRECTION('',(0.,-1.,0.));
#4792=DIRECTION('center_axis',(0.,1.,0.));
#4793=DIRECTION('ref_axis',(0.,0.,1.));
#4794=DIRECTION('center_axis',(0.,-1.,0.));
#4795=DIRECTION('ref_axis',(0.,0.,-1.));
#4796=DIRECTION('center_axis',(0.,1.,0.));
#4797=DIRECTION('ref_axis',(0.,0.,1.));
#4798=DIRECTION('center_axis',(0.,-1.,0.));
#4799=DIRECTION('ref_axis',(0.,0.,-1.));
#4800=DIRECTION('',(0.,-1.,0.));
#4801=DIRECTION('center_axis',(0.,1.,0.));
#4802=DIRECTION('ref_axis',(0.,0.,1.));
#4803=DIRECTION('',(0.,1.,0.));
#4804=DIRECTION('center_axis',(0.,1.,0.));
#4805=DIRECTION('ref_axis',(0.,0.,1.));
#4806=DIRECTION('',(0.,-1.,0.));
#4807=DIRECTION('center_axis',(0.,-1.,0.));
#4808=DIRECTION('ref_axis',(0.,0.,-1.));
#4809=DIRECTION('',(0.,-1.,0.));
#4810=DIRECTION('center_axis',(0.,1.,0.));
#4811=DIRECTION('ref_axis',(0.,0.,1.));
#4812=DIRECTION('',(0.,-1.,0.));
#4813=DIRECTION('center_axis',(0.,-1.,0.));
#4814=DIRECTION('ref_axis',(0.,0.,-1.));
#4815=DIRECTION('center_axis',(0.,1.,0.));
#4816=DIRECTION('ref_axis',(0.,0.,1.));
#4817=DIRECTION('center_axis',(0.,-1.,0.));
#4818=DIRECTION('ref_axis',(0.,0.,-1.));
#4819=DIRECTION('',(0.,0.,1.));
#4820=DIRECTION('',(0.,0.,1.));
#4821=DIRECTION('center_axis',(0.,-1.,0.));
#4822=DIRECTION('ref_axis',(0.,0.,-1.));
#4823=DIRECTION('center_axis',(0.,-1.,0.));
#4824=DIRECTION('ref_axis',(0.,0.,-1.));
#4825=DIRECTION('center_axis',(0.,-1.,0.));
#4826=DIRECTION('ref_axis',(0.,0.,-1.));
#4827=DIRECTION('',(0.,1.,0.));
#4828=DIRECTION('center_axis',(0.,1.,0.));
#4829=DIRECTION('ref_axis',(0.,0.,1.));
#4830=DIRECTION('',(8.65956056235493E-17,-0.707106781186548,0.707106781186547));
#4831=DIRECTION('center_axis',(0.,-1.,0.));
#4832=DIRECTION('ref_axis',(1.,0.,3.49148133884313E-15));
#4833=DIRECTION('center_axis',(0.,-1.,0.));
#4834=DIRECTION('ref_axis',(0.,0.,-1.));
#4835=DIRECTION('center_axis',(0.,-1.,0.));
#4836=DIRECTION('ref_axis',(1.,0.,3.49148133884313E-15));
#4837=DIRECTION('center_axis',(0.,-1.,0.));
#4838=DIRECTION('ref_axis',(0.,0.,-1.));
#4839=DIRECTION('center_axis',(0.,-1.,0.));
#4840=DIRECTION('ref_axis',(1.,0.,3.49148133884313E-15));
#4841=DIRECTION('center_axis',(-1.,0.,0.));
#4842=DIRECTION('ref_axis',(0.,0.,1.));
#4843=DIRECTION('',(0.,0.,1.));
#4844=DIRECTION('center_axis',(0.,1.,0.));
#4845=DIRECTION('ref_axis',(0.,0.,1.));
#4846=DIRECTION('',(0.,0.,1.));
#4847=DIRECTION('center_axis',(0.,1.,0.));
#4848=DIRECTION('ref_axis',(0.,0.,1.));
#4849=DIRECTION('center_axis',(1.,0.,0.));
#4850=DIRECTION('ref_axis',(0.,0.,-1.));
#4851=DIRECTION('center_axis',(0.,-1.,0.));
#4852=DIRECTION('ref_axis',(0.,0.,-1.));
#4853=DIRECTION('',(0.,-1.,0.));
#4854=DIRECTION('center_axis',(0.,1.,0.));
#4855=DIRECTION('ref_axis',(0.,0.,1.));
#4856=DIRECTION('center_axis',(0.,-1.,0.));
#4857=DIRECTION('ref_axis',(0.,0.,-1.));
#4858=DIRECTION('center_axis',(0.,1.,0.));
#4859=DIRECTION('ref_axis',(0.,0.,1.));
#4860=DIRECTION('center_axis',(0.,-1.,0.));
#4861=DIRECTION('ref_axis',(0.,0.,-1.));
#4862=DIRECTION('center_axis',(0.,-1.,0.));
#4863=DIRECTION('ref_axis',(0.,0.,-1.));
#4864=DIRECTION('',(-3.48532219369785E-15,0.,1.));
#4865=DIRECTION('center_axis',(0.,-1.,0.));
#4866=DIRECTION('ref_axis',(0.,0.,-1.));
#4867=DIRECTION('',(3.48532219369785E-15,0.,-1.));
#4868=DIRECTION('center_axis',(0.,-1.,0.));
#4869=DIRECTION('ref_axis',(0.,0.,-1.));
#4870=DIRECTION('',(3.51320477124743E-15,0.,-1.));
#4871=DIRECTION('center_axis',(0.,-1.,0.));
#4872=DIRECTION('ref_axis',(0.,0.,-1.));
#4873=DIRECTION('',(-3.49926348247264E-15,0.,1.));
#4874=DIRECTION('center_axis',(0.,-1.,0.));
#4875=DIRECTION('ref_axis',(0.,0.,-1.));
#4876=DIRECTION('center_axis',(-1.,0.,-3.49148133884313E-15));
#4877=DIRECTION('ref_axis',(-3.49148133884313E-15,0.,1.));
#4878=DIRECTION('',(0.,1.,0.));
#4879=DIRECTION('center_axis',(1.,0.,3.49148133884313E-15));
#4880=DIRECTION('ref_axis',(3.49148133884313E-15,0.,-1.));
#4881=DIRECTION('',(0.,1.,0.));
#4882=DIRECTION('center_axis',(0.,1.,0.));
#4883=DIRECTION('ref_axis',(3.67517835871524E-15,0.,-1.));
#4884=DIRECTION('center_axis',(0.,-1.,0.));
#4885=DIRECTION('ref_axis',(0.,0.,-1.));
#4886=DIRECTION('center_axis',(1.,0.,3.49148133884313E-15));
#4887=DIRECTION('ref_axis',(3.49148133884313E-15,0.,-1.));
#4888=DIRECTION('',(0.,1.,0.));
#4889=DIRECTION('center_axis',(-1.,0.,-3.49148133884313E-15));
#4890=DIRECTION('ref_axis',(-3.49148133884313E-15,0.,1.));
#4891=DIRECTION('',(0.,1.,0.));
#4892=DIRECTION('center_axis',(0.,1.,0.));
#4893=DIRECTION('ref_axis',(0.,0.,1.));
#4894=DIRECTION('center_axis',(0.,-1.,0.));
#4895=DIRECTION('ref_axis',(0.,0.,-1.));
#4896=DIRECTION('center_axis',(0.,1.,0.));
#4897=DIRECTION('ref_axis',(0.,0.,1.));
#4898=DIRECTION('center_axis',(0.,1.,0.));
#4899=DIRECTION('ref_axis',(0.,0.,1.));
#4900=DIRECTION('center_axis',(0.,1.,0.));
#4901=DIRECTION('ref_axis',(3.43024899888577E-15,0.,-1.));
#4902=DIRECTION('center_axis',(0.,1.,0.));
#4903=DIRECTION('ref_axis',(0.,0.,1.));
#6258=CARTESIAN_POINT('',(0.,0.,0.));
#6259=CARTESIAN_POINT('Origin',(26.,0.,0.));
#6260=CARTESIAN_POINT('',(-25.9229627936314,0.,-2.));
#6261=CARTESIAN_POINT('',(-1.99999999999991,0.,-25.9229627936314));
#6262=CARTESIAN_POINT('Origin',(0.,0.,0.));
#6263=CARTESIAN_POINT('',(-2.,0.,-2.));
#6264=CARTESIAN_POINT('',(-1.99999999999999,0.,-2.));
#6265=CARTESIAN_POINT('',(-25.9229627936314,0.,-2.));
#6266=CARTESIAN_POINT('Origin',(26.,0.,0.));
#6267=CARTESIAN_POINT('',(2.00000000000001,0.,-2.));
#6268=CARTESIAN_POINT('',(25.9229627936314,0.,-2.));
#6269=CARTESIAN_POINT('',(2.00000000000001,0.,-2.));
#6270=CARTESIAN_POINT('',(2.00000000000009,0.,-25.9229627936314));
#6271=CARTESIAN_POINT('',(2.00000000000009,0.,-25.9229627936314));
#6272=CARTESIAN_POINT('Origin',(0.,0.,0.));
#6273=CARTESIAN_POINT('Origin',(26.,0.,0.));
#6274=CARTESIAN_POINT('',(-2.00000000000001,0.,2.));
#6275=CARTESIAN_POINT('',(-25.9229627936314,0.,2.));
#6276=CARTESIAN_POINT('',(-2.00000000000001,0.,2.));
#6277=CARTESIAN_POINT('',(-2.00000000000009,0.,25.9229627936314));
#6278=CARTESIAN_POINT('',(-2.00000000000009,0.,25.9229627936314));
#6279=CARTESIAN_POINT('Origin',(0.,0.,0.));
#6280=CARTESIAN_POINT('Origin',(26.,0.,0.));
#6281=CARTESIAN_POINT('',(25.9229627936314,0.,2.));
#6282=CARTESIAN_POINT('',(1.99999999999991,0.,25.9229627936315));
#6283=CARTESIAN_POINT('Origin',(0.,0.,0.));
#6284=CARTESIAN_POINT('',(2.,0.,2.));
#6285=CARTESIAN_POINT('',(1.99999999999999,0.,2.));
#6286=CARTESIAN_POINT('',(25.9229627936314,0.,2.));
#6287=CARTESIAN_POINT('Origin',(-25.9229627936314,-24.,2.));
#6288=CARTESIAN_POINT('',(-25.9229627936314,-20.,2.));
#6289=CARTESIAN_POINT('',(-25.9229627936314,-20.,2.));
#6290=CARTESIAN_POINT('',(-21.9089023002066,-24.,2.));
#6291=CARTESIAN_POINT('Ctrl Pts',(-25.9229627936293,-20.0000000000019,2.));
#6292=CARTESIAN_POINT('Ctrl Pts',(-23.7486800263697,-22.1678404337906,2.));
#6293=CARTESIAN_POINT('Ctrl Pts',(-21.9089023002066,-24.,2.));
#6294=CARTESIAN_POINT('',(-2.,-24.,2.));
#6295=CARTESIAN_POINT('',(-2.,-24.,2.));
#6296=CARTESIAN_POINT('',(-2.00000000000002,0.,2.));
#6297=CARTESIAN_POINT('Origin',(-25.9229627936314,-24.,2.));
#6298=CARTESIAN_POINT('',(21.9089023002066,-24.,2.));
#6299=CARTESIAN_POINT('',(1.99999999999999,-24.,2.));
#6300=CARTESIAN_POINT('',(21.9089023002066,-24.,2.));
#6301=CARTESIAN_POINT('',(25.9229627936314,-20.,2.));
#6302=CARTESIAN_POINT('Ctrl Pts',(21.9089023002321,-23.9999999999746,2.));
#6303=CARTESIAN_POINT('Ctrl Pts',(23.7486800263847,-22.1678404337756,2.));
#6304=CARTESIAN_POINT('Ctrl Pts',(25.9229627936293,-20.0000000000019,2.));
#6305=CARTESIAN_POINT('',(25.9229627936314,-20.,2.));
#6306=CARTESIAN_POINT('',(1.99999999999998,-24.,2.));
#6307=CARTESIAN_POINT('Origin',(-25.9229627936314,-24.,-2.));
#6308=CARTESIAN_POINT('',(-21.9089023002066,-24.,-2.));
#6309=CARTESIAN_POINT('',(-1.99999999999999,-24.,-2.));
#6310=CARTESIAN_POINT('',(-21.9089023002066,-24.,-2.));
#6311=CARTESIAN_POINT('',(-25.9229627936314,-20.,-2.));
#6312=CARTESIAN_POINT('Ctrl Pts',(-21.9089023002321,-23.9999999999746,-2.));
#6313=CARTESIAN_POINT('Ctrl Pts',(-23.7486800263847,-22.1678404337756,-2.));
#6314=CARTESIAN_POINT('Ctrl Pts',(-25.9229627936293,-20.0000000000019,-2.));
#6315=CARTESIAN_POINT('',(-25.9229627936314,-20.,-2.));
#6316=CARTESIAN_POINT('',(-1.99999999999998,-24.,-2.));
#6317=CARTESIAN_POINT('Origin',(-25.9229627936314,-24.,-2.));
#6318=CARTESIAN_POINT('',(25.9229627936314,-20.,-2.));
#6319=CARTESIAN_POINT('',(25.9229627936314,-20.,-2.));
#6320=CARTESIAN_POINT('',(21.9089023002066,-24.,-2.));
#6321=CARTESIAN_POINT('Ctrl Pts',(25.9229627936293,-20.0000000000019,-2.));
#6322=CARTESIAN_POINT('Ctrl Pts',(23.7486800263697,-22.1678404337906,-2.));
#6323=CARTESIAN_POINT('Ctrl Pts',(21.9089023002066,-24.,-2.));
#6324=CARTESIAN_POINT('',(2.,-24.,-2.));
#6325=CARTESIAN_POINT('',(2.,-24.,-2.));
#6326=CARTESIAN_POINT('',(2.00000000000002,0.,-2.));
#6327=CARTESIAN_POINT('Origin',(0.,30.,0.));
#6328=CARTESIAN_POINT('',(-2.93915231795365E-15,30.,24.));
#6329=CARTESIAN_POINT('Origin',(0.,30.,0.));
#6330=CARTESIAN_POINT('',(0.,30.,11.));
#6331=CARTESIAN_POINT('Origin',(0.,30.,0.));
#6332=CARTESIAN_POINT('Origin',(0.,0.,0.));
#6333=CARTESIAN_POINT('',(-16.,24.,17.8885438199983));
#6334=CARTESIAN_POINT('',(-16.,8.,17.8885438199983));
#6335=CARTESIAN_POINT('',(-16.,24.,17.8885438199983));
#6336=CARTESIAN_POINT('',(-2.93915231795365E-15,24.,24.));
#6337=CARTESIAN_POINT('Origin',(0.,24.,0.));
#6338=CARTESIAN_POINT('',(-2.93915231795365E-15,0.,24.));
#6339=CARTESIAN_POINT('',(16.,24.,17.8885438199983));
#6340=CARTESIAN_POINT('Origin',(0.,24.,0.));
#6341=CARTESIAN_POINT('',(16.,8.,17.8885438199983));
#6342=CARTESIAN_POINT('',(16.,24.,17.8885438199983));
#6343=CARTESIAN_POINT('',(16.,8.,-17.8885438199983));
#6344=CARTESIAN_POINT('Origin',(0.,8.,0.));
#6345=CARTESIAN_POINT('',(16.,24.,-17.8885438199983));
#6346=CARTESIAN_POINT('',(16.,24.,-17.8885438199983));
#6347=CARTESIAN_POINT('',(-16.,24.,-17.8885438199983));
#6348=CARTESIAN_POINT('Origin',(0.,24.,0.));
#6349=CARTESIAN_POINT('',(-16.,8.,-17.8885438199983));
#6350=CARTESIAN_POINT('',(-16.,24.,-17.8885438199983));
#6351=CARTESIAN_POINT('Origin',(0.,8.,0.));
#6352=CARTESIAN_POINT('Origin',(24.,8.,0.));
#6353=CARTESIAN_POINT('',(-3.67394039744206E-15,8.,30.));
#6354=CARTESIAN_POINT('Origin',(0.,8.,0.));
#6355=CARTESIAN_POINT('',(16.,8.,-17.8885438199983));
#6356=CARTESIAN_POINT('',(-16.,8.,-17.8885438199983));
#6357=CARTESIAN_POINT('Origin',(0.,0.,0.));
#6358=CARTESIAN_POINT('',(0.,4.,-30.));
#6359=CARTESIAN_POINT('',(-3.67394039744206E-15,4.,30.));
#6360=CARTESIAN_POINT('Origin',(0.,4.,0.));
#6361=CARTESIAN_POINT('Origin',(0.,4.,0.));
#6362=CARTESIAN_POINT('',(-3.67394039744206E-15,0.,30.));
#6363=CARTESIAN_POINT('Origin',(0.,0.,0.));
#6364=CARTESIAN_POINT('',(-3.18408167778312E-15,-2.35143570712168E-15,-26.));
#6365=CARTESIAN_POINT('',(-3.18408167778312E-15,0.,-26.));
#6366=CARTESIAN_POINT('Origin',(0.,0.,0.));
#6367=CARTESIAN_POINT('Origin',(0.,0.,0.));
#6368=CARTESIAN_POINT('Origin',(0.,0.,0.));
#6369=CARTESIAN_POINT('Origin',(0.,0.,0.));
#6370=CARTESIAN_POINT('Origin',(0.,0.,0.));
#6371=CARTESIAN_POINT('Origin',(-16.,8.,-30.));
#6372=CARTESIAN_POINT('',(-16.,24.,-17.8885438199983));
#6373=CARTESIAN_POINT('Origin',(-16.,24.,-30.));
#6374=CARTESIAN_POINT('',(16.,24.,-17.8885438199983));
#6375=CARTESIAN_POINT('',(0.,24.,11.));
#6376=CARTESIAN_POINT('Origin',(0.,24.,0.));
#6377=CARTESIAN_POINT('Origin',(16.,8.,-30.));
#6378=CARTESIAN_POINT('Origin',(0.,30.000012,0.));
#6379=CARTESIAN_POINT('',(-1.34711147906209E-15,30.000012,11.));
#6380=CARTESIAN_POINT('Origin',(0.,-24.,0.));
#6381=CARTESIAN_POINT('Origin',(0.,-20.,0.));
#6382=CARTESIAN_POINT('Origin',(0.,-24.,0.));
#6383=CARTESIAN_POINT('Origin',(0.,-20.,0.));
#6384=CARTESIAN_POINT('Origin',(0.,-24.,0.));
#6385=CARTESIAN_POINT('',(1.99999999999992,-24.,21.9089023002066));
#6386=CARTESIAN_POINT('',(1.99999999999999,-24.,2.));
#6387=CARTESIAN_POINT('',(-2.00000000000008,-24.,21.9089023002066));
#6388=CARTESIAN_POINT('Origin',(0.,-24.,0.));
#6389=CARTESIAN_POINT('',(-2.00000000000008,-24.,21.9089023002066));
#6390=CARTESIAN_POINT('Origin',(0.,-24.,0.));
#6391=CARTESIAN_POINT('',(-1.99999999999992,-24.,-21.9089023002066));
#6392=CARTESIAN_POINT('',(-1.99999999999999,-24.,-2.));
#6393=CARTESIAN_POINT('',(2.00000000000008,-24.,-21.9089023002066));
#6394=CARTESIAN_POINT('Origin',(0.,-24.,0.));
#6395=CARTESIAN_POINT('',(2.00000000000008,-24.,-21.9089023002066));
#6396=CARTESIAN_POINT('Origin',(0.,-24.,0.));
#6397=CARTESIAN_POINT('Origin',(2.00000000000009,-24.,-25.9229627936314));
#6398=CARTESIAN_POINT('',(2.00000000000009,-20.,-25.9229627936314));
#6399=CARTESIAN_POINT('Ctrl Pts',(2.00000000000008,-23.9999999999746,-21.9089023002321));
#6400=CARTESIAN_POINT('Ctrl Pts',(2.00000000000008,-22.1678404337738,-23.7486800263865));
#6401=CARTESIAN_POINT('Ctrl Pts',(2.00000000000009,-20.0000000000019,-25.9229627936293));
#6402=CARTESIAN_POINT('',(2.00000000000009,-20.,-25.9229627936314));
#6403=CARTESIAN_POINT('Origin',(-1.99999999999991,-24.,-25.9229627936314));
#6404=CARTESIAN_POINT('',(-1.99999999999991,-20.,-25.9229627936314));
#6405=CARTESIAN_POINT('',(-1.99999999999991,-20.,-25.9229627936314));
#6406=CARTESIAN_POINT('Ctrl Pts',(-1.99999999999991,-20.0000000000021,-25.9229627936295));
#6407=CARTESIAN_POINT('Ctrl Pts',(-1.99999999999992,-22.167840433814,-23.7486800263466));
#6408=CARTESIAN_POINT('Ctrl Pts',(-1.99999999999992,-24.,-21.9089023002067));
#6409=CARTESIAN_POINT('Origin',(0.,-24.,0.));
#6410=CARTESIAN_POINT('Origin',(0.,-20.,0.));
#6411=CARTESIAN_POINT('Origin',(-1.99999999999991,-24.,-25.9229627936314));
#6412=CARTESIAN_POINT('',(-2.00000000000009,-20.,25.9229627936314));
#6413=CARTESIAN_POINT('Ctrl Pts',(-2.00000000000008,-23.9999999999746,21.9089023002321));
#6414=CARTESIAN_POINT('Ctrl Pts',(-2.00000000000008,-22.1678404337738,23.7486800263865));
#6415=CARTESIAN_POINT('Ctrl Pts',(-2.00000000000009,-20.0000000000019,25.9229627936293));
#6416=CARTESIAN_POINT('',(-2.00000000000009,-20.,25.9229627936314));
#6417=CARTESIAN_POINT('Origin',(2.00000000000009,-24.,-25.9229627936314));
#6418=CARTESIAN_POINT('',(1.99999999999991,-20.,25.9229627936315));
#6419=CARTESIAN_POINT('',(1.99999999999991,-20.,25.9229627936315));
#6420=CARTESIAN_POINT('Ctrl Pts',(1.99999999999991,-20.0000000000021,25.9229627936295));
#6421=CARTESIAN_POINT('Ctrl Pts',(1.99999999999992,-22.1678404338147,23.7486800263459));
#6422=CARTESIAN_POINT('Ctrl Pts',(1.99999999999992,-24.,21.9089023002067));
#6423=CARTESIAN_POINT('Origin',(0.,-24.,0.));
#6424=CARTESIAN_POINT('Origin',(0.,-20.,0.));
#6425=CARTESIAN_POINT('Origin',(0.,-24.,0.));
#6426=CARTESIAN_POINT('Origin',(0.,-24.,0.));
#6427=CARTESIAN_POINT('Origin',(0.,-24.,0.));
#6428=CARTESIAN_POINT('Origin',(0.,-24.,0.));
#9645=UNCERTAINTY_MEASURE_WITH_UNIT(LENGTH_MEASURE(0.01),#9669,
'DISTANCE_ACCURACY_VALUE',
'Maximum model space distance between geometric entities at asserted c
onnectivities');
#9655=UNCERTAINTY_MEASURE_WITH_UNIT(LENGTH_MEASURE(0.01),#9669,
'DISTANCE_ACCURACY_VALUE',
'Maximum model space distance between geometric entities at asserted c
onnectivities');
#9658=(
GEOMETRIC_REPRESENTATION_CONTEXT(3)
GLOBAL_UNCERTAINTY_ASSIGNED_CONTEXT((#9645))
GLOBAL_UNIT_ASSIGNED_CONTEXT((#9669,#9671,#9672))
REPRESENTATION_CONTEXT('','3D')
);
#9668=(
GEOMETRIC_REPRESENTATION_CONTEXT(3)
GLOBAL_UNCERTAINTY_ASSIGNED_CONTEXT((#9655))
GLOBAL_UNIT_ASSIGNED_CONTEXT((#9669,#9671,#9672))
REPRESENTATION_CONTEXT('','3D')
);
#9669=(
LENGTH_UNIT()
NAMED_UNIT(*)
SI_UNIT(.MILLI.,.METRE.)
);
#9671=(
NAMED_UNIT(*)
PLANE_ANGLE_UNIT()
SI_UNIT($,.RADIAN.)
);
#9672=(
NAMED_UNIT(*)
SI_UNIT($,.STERADIAN.)
SOLID_ANGLE_UNIT()
);
#9675=SHAPE_DEFINITION_REPRESENTATION(#9687,#9713);
#9687=PRODUCT_DEFINITION_SHAPE('',$,#9726);
#9713=SHAPE_REPRESENTATION('',(#4135),#9658);
#9723=PRODUCT_DEFINITION_CONTEXT('part definition',#9761,'design');
#9726=PRODUCT_DEFINITION('2026-10-04-08-13-48-881','VALVE_DISC',#9738,#9723);
#9738=PRODUCT_DEFINITION_FORMATION('',$,#9765);
#9761=APPLICATION_CONTEXT(
'Core Data for Automotive Mechanical Design Process');
#9762=PRODUCT_CONTEXT('part definition',#9761,'mechanical');
#9765=PRODUCT('2026-10-04-08-13-48-881','VALVE_DISC','PART',(#9762));
#9775=PRESENTATION_STYLE_ASSIGNMENT((#9776));
#9776=SURFACE_STYLE_USAGE(.BOTH.,#9777);
#9777=SURFACE_SIDE_STYLE('',(#9778));
#9778=SURFACE_STYLE_FILL_AREA(#9779);
#9779=FILL_AREA_STYLE('Steel - Satin',(#9780));
#9780=FILL_AREA_STYLE_COLOUR('Steel - Satin',#9781);
#9781=COLOUR_RGB('Steel - Satin', 0.09019608, 0.27058824, 0.51372549);
ENDSEC;
END-ISO-10303-21;
